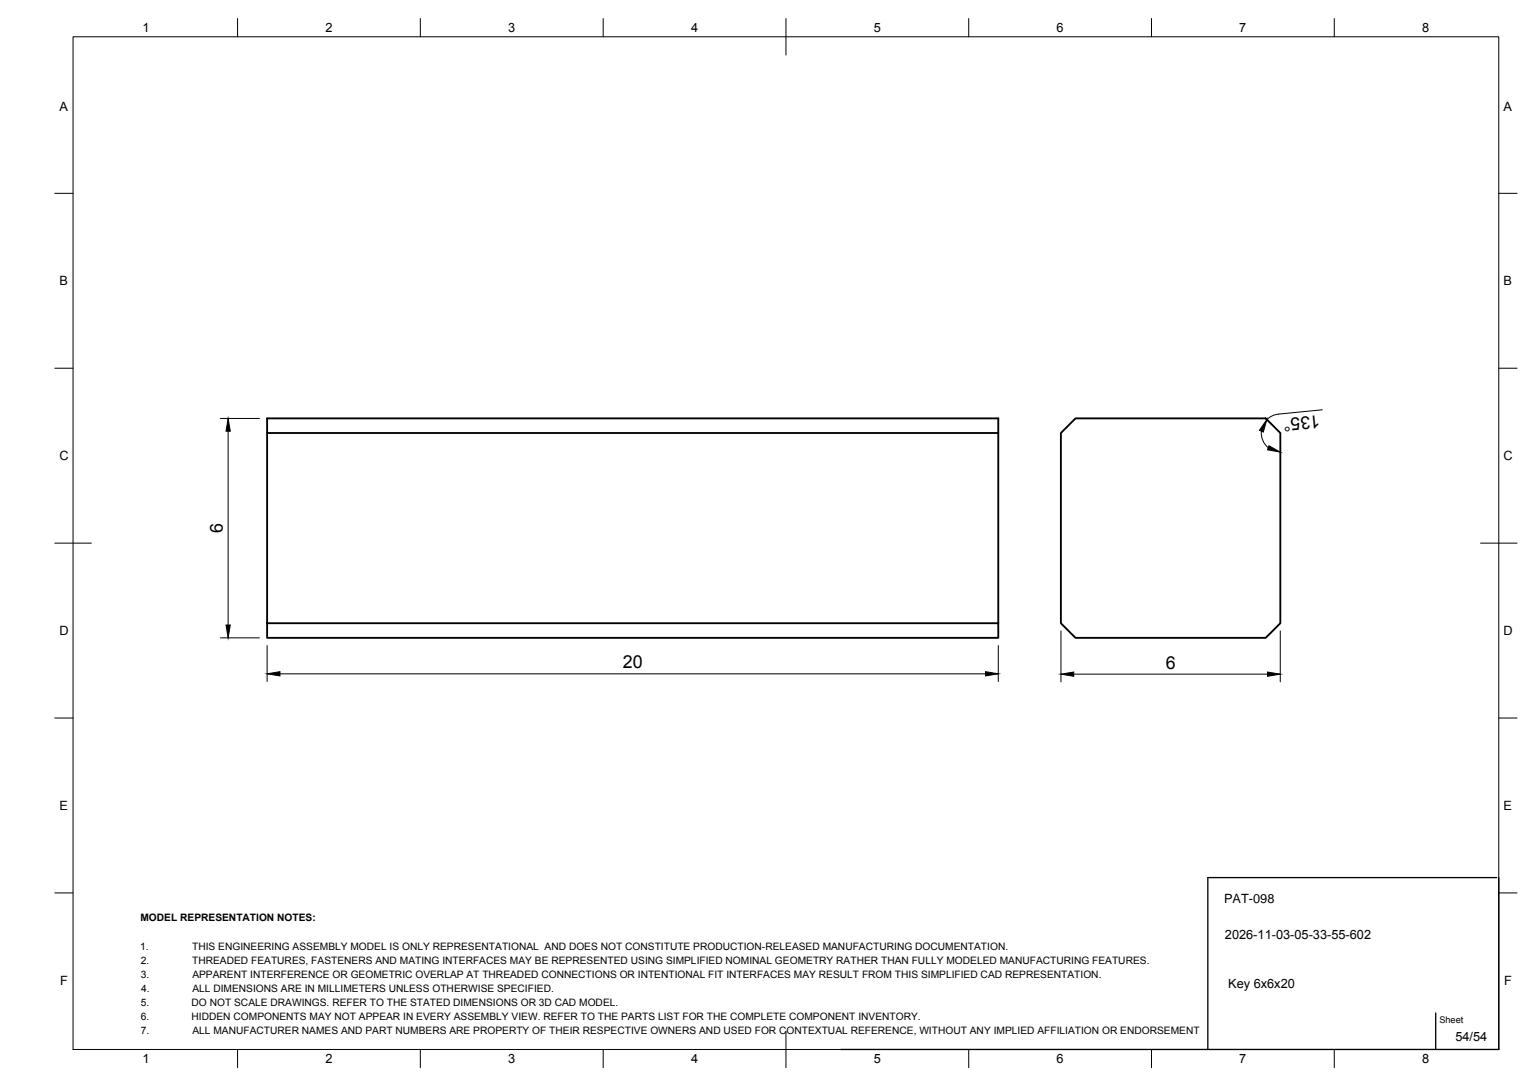
ISO-10303-21;
HEADER;
/* Generated by software containing ST-Developer
 * from STEP Tools, Inc. (www.steptools.com) 
 */

FILE_DESCRIPTION(
/* description */ ('Spring compression tester'),
/* implementation_level */ '2;1');

FILE_NAME(
/* name */ 'Key 6x6x20.step',
/* time_stamp */ '2026-10-28T03:24:11-07:00',
/* author */ (''),
/* organization */ (''),
/* preprocessor_version */ 'ST-DEVELOPER v20.2',
/* originating_system */ 'Autodesk Translation Framework v15.17.0.0',
/* authorisation */ '');

FILE_SCHEMA (('AUTOMOTIVE_DESIGN { 1 0 10303 214 3 1 1 }'));
ENDSEC;

DATA;
#10=MECHANICAL_DESIGN_GEOMETRIC_PRESENTATION_REPRESENTATION('',(#1175),#43521);
#1040=SHAPE_REPRESENTATION_RELATIONSHIP('SRR','None',#43857,#1100);
#1100=ADVANCED_BREP_SHAPE_REPRESENTATION('',(#1244),#43517);
#1175=STYLED_ITEM('',(#44202),#1244);
#1244=MANIFOLD_SOLID_BREP('Body1',#18618);
#2138=PLANE('',#21120);
#2139=PLANE('',#21121);
#2140=PLANE('',#21122);
#2141=PLANE('',#21123);
#2142=PLANE('',#21124);
#2143=PLANE('',#21125);
#2144=PLANE('',#21126);
#2145=PLANE('',#21127);
#2146=PLANE('',#21128);
#2147=PLANE('',#21129);
#3174=FACE_OUTER_BOUND('',#4559,.T.);
#3175=FACE_OUTER_BOUND('',#4560,.T.);
#3176=FACE_OUTER_BOUND('',#4561,.T.);
#3177=FACE_OUTER_BOUND('',#4562,.T.);
#3178=FACE_OUTER_BOUND('',#4563,.T.);
#3179=FACE_OUTER_BOUND('',#4564,.T.);
#3180=FACE_OUTER_BOUND('',#4565,.T.);
#3181=FACE_OUTER_BOUND('',#4566,.T.);
#3182=FACE_OUTER_BOUND('',#4567,.T.);
#3183=FACE_OUTER_BOUND('',#4568,.T.);
#4559=EDGE_LOOP('',(#16931,#16932,#16933,#16934,#16935,#16936,#16937,#16938));
#4560=EDGE_LOOP('',(#16939,#16940,#16941,#16942));
#4561=EDGE_LOOP('',(#16943,#16944,#16945,#16946));
#4562=EDGE_LOOP('',(#16947,#16948,#16949,#16950));
#4563=EDGE_LOOP('',(#16951,#16952,#16953,#16954));
#4564=EDGE_LOOP('',(#16955,#16956,#16957,#16958,#16959,#16960,#16961,#16962));
#4565=EDGE_LOOP('',(#16963,#16964,#16965,#16966));
#4566=EDGE_LOOP('',(#16967,#16968,#16969,#16970));
#4567=EDGE_LOOP('',(#16971,#16972,#16973,#16974));
#4568=EDGE_LOOP('',(#16975,#16976,#16977,#16978));
#5967=LINE('',#43186,#7399);
#5968=LINE('',#43188,#7400);
#5969=LINE('',#43190,#7401);
#5970=LINE('',#43192,#7402);
#5971=LINE('',#43194,#7403);
#5972=LINE('',#43196,#7404);
#5973=LINE('',#43198,#7405);
#5974=LINE('',#43199,#7406);
#5975=LINE('',#43202,#7407);
#5976=LINE('',#43204,#7408);
#5977=LINE('',#43205,#7409);
#5978=LINE('',#43208,#7410);
#5979=LINE('',#43209,#7411);
#5980=LINE('',#43212,#7412);
#5981=LINE('',#43213,#7413);
#5982=LINE('',#43216,#7414);
#5983=LINE('',#43217,#7415);
#5984=LINE('',#43221,#7416);
#5985=LINE('',#43222,#7417);
#5986=LINE('',#43224,#7418);
#5987=LINE('',#43225,#7419);
#5988=LINE('',#43227,#7420);
#5989=LINE('',#43229,#7421);
#5990=LINE('',#43231,#7422);
#7399=VECTOR('',#26231,1.);
#7400=VECTOR('',#26232,1.);
#7401=VECTOR('',#26233,1.);
#7402=VECTOR('',#26234,1.);
#7403=VECTOR('',#26235,1.);
#7404=VECTOR('',#26236,1.);
#7405=VECTOR('',#26237,1.);
#7406=VECTOR('',#26238,1.);
#7407=VECTOR('',#26241,1.);
#7408=VECTOR('',#26242,1.);
#7409=VECTOR('',#26243,1.);
#7410=VECTOR('',#26246,1.);
#7411=VECTOR('',#26247,1.);
#7412=VECTOR('',#26250,1.);
#7413=VECTOR('',#26251,1.);
#7414=VECTOR('',#26254,1.);
#7415=VECTOR('',#26255,1.);
#7416=VECTOR('',#26258,1.);
#7417=VECTOR('',#26259,1.);
#7418=VECTOR('',#26260,1.);
#7419=VECTOR('',#26261,1.);
#7420=VECTOR('',#26264,1.);
#7421=VECTOR('',#26267,1.);
#7422=VECTOR('',#26270,1.);
#9717=VERTEX_POINT('',#43184);
#9718=VERTEX_POINT('',#43185);
#9719=VERTEX_POINT('',#43187);
#9720=VERTEX_POINT('',#43189);
#9721=VERTEX_POINT('',#43191);
#9722=VERTEX_POINT('',#43193);
#9723=VERTEX_POINT('',#43195);
#9724=VERTEX_POINT('',#43197);
#9725=VERTEX_POINT('',#43201);
#9726=VERTEX_POINT('',#43203);
#9727=VERTEX_POINT('',#43207);
#9728=VERTEX_POINT('',#43211);
#9729=VERTEX_POINT('',#43215);
#9730=VERTEX_POINT('',#43219);
#9731=VERTEX_POINT('',#43220);
#9732=VERTEX_POINT('',#43223);
#12130=EDGE_CURVE('',#9717,#9718,#5967,.T.);
#12131=EDGE_CURVE('',#9719,#9717,#5968,.T.);
#12132=EDGE_CURVE('',#9720,#9719,#5969,.T.);
#12133=EDGE_CURVE('',#9721,#9720,#5970,.T.);
#12134=EDGE_CURVE('',#9722,#9721,#5971,.T.);
#12135=EDGE_CURVE('',#9723,#9722,#5972,.T.);
#12136=EDGE_CURVE('',#9724,#9723,#5973,.T.);
#12137=EDGE_CURVE('',#9718,#9724,#5974,.T.);
#12138=EDGE_CURVE('',#9721,#9725,#5975,.T.);
#12139=EDGE_CURVE('',#9725,#9726,#5976,.T.);
#12140=EDGE_CURVE('',#9726,#9722,#5977,.T.);
#12141=EDGE_CURVE('',#9727,#9720,#5978,.T.);
#12142=EDGE_CURVE('',#9727,#9725,#5979,.T.);
#12143=EDGE_CURVE('',#9719,#9728,#5980,.T.);
#12144=EDGE_CURVE('',#9728,#9727,#5981,.T.);
#12145=EDGE_CURVE('',#9729,#9717,#5982,.T.);
#12146=EDGE_CURVE('',#9729,#9728,#5983,.T.);
#12147=EDGE_CURVE('',#9730,#9731,#5984,.T.);
#12148=EDGE_CURVE('',#9726,#9730,#5985,.T.);
#12149=EDGE_CURVE('',#9732,#9729,#5986,.T.);
#12150=EDGE_CURVE('',#9731,#9732,#5987,.T.);
#12151=EDGE_CURVE('',#9723,#9730,#5988,.T.);
#12152=EDGE_CURVE('',#9718,#9732,#5989,.T.);
#12153=EDGE_CURVE('',#9731,#9724,#5990,.T.);
#16931=ORIENTED_EDGE('',*,*,#12130,.F.);
#16932=ORIENTED_EDGE('',*,*,#12131,.F.);
#16933=ORIENTED_EDGE('',*,*,#12132,.F.);
#16934=ORIENTED_EDGE('',*,*,#12133,.F.);
#16935=ORIENTED_EDGE('',*,*,#12134,.F.);
#16936=ORIENTED_EDGE('',*,*,#12135,.F.);
#16937=ORIENTED_EDGE('',*,*,#12136,.F.);
#16938=ORIENTED_EDGE('',*,*,#12137,.F.);
#16939=ORIENTED_EDGE('',*,*,#12134,.T.);
#16940=ORIENTED_EDGE('',*,*,#12138,.T.);
#16941=ORIENTED_EDGE('',*,*,#12139,.T.);
#16942=ORIENTED_EDGE('',*,*,#12140,.T.);
#16943=ORIENTED_EDGE('',*,*,#12133,.T.);
#16944=ORIENTED_EDGE('',*,*,#12141,.F.);
#16945=ORIENTED_EDGE('',*,*,#12142,.T.);
#16946=ORIENTED_EDGE('',*,*,#12138,.F.);
#16947=ORIENTED_EDGE('',*,*,#12132,.T.);
#16948=ORIENTED_EDGE('',*,*,#12143,.T.);
#16949=ORIENTED_EDGE('',*,*,#12144,.T.);
#16950=ORIENTED_EDGE('',*,*,#12141,.T.);
#16951=ORIENTED_EDGE('',*,*,#12131,.T.);
#16952=ORIENTED_EDGE('',*,*,#12145,.F.);
#16953=ORIENTED_EDGE('',*,*,#12146,.T.);
#16954=ORIENTED_EDGE('',*,*,#12143,.F.);
#16955=ORIENTED_EDGE('',*,*,#12147,.F.);
#16956=ORIENTED_EDGE('',*,*,#12148,.F.);
#16957=ORIENTED_EDGE('',*,*,#12139,.F.);
#16958=ORIENTED_EDGE('',*,*,#12142,.F.);
#16959=ORIENTED_EDGE('',*,*,#12144,.F.);
#16960=ORIENTED_EDGE('',*,*,#12146,.F.);
#16961=ORIENTED_EDGE('',*,*,#12149,.F.);
#16962=ORIENTED_EDGE('',*,*,#12150,.F.);
#16963=ORIENTED_EDGE('',*,*,#12135,.T.);
#16964=ORIENTED_EDGE('',*,*,#12140,.F.);
#16965=ORIENTED_EDGE('',*,*,#12148,.T.);
#16966=ORIENTED_EDGE('',*,*,#12151,.F.);
#16967=ORIENTED_EDGE('',*,*,#12130,.T.);
#16968=ORIENTED_EDGE('',*,*,#12152,.T.);
#16969=ORIENTED_EDGE('',*,*,#12149,.T.);
#16970=ORIENTED_EDGE('',*,*,#12145,.T.);
#16971=ORIENTED_EDGE('',*,*,#12136,.T.);
#16972=ORIENTED_EDGE('',*,*,#12151,.T.);
#16973=ORIENTED_EDGE('',*,*,#12147,.T.);
#16974=ORIENTED_EDGE('',*,*,#12153,.T.);
#16975=ORIENTED_EDGE('',*,*,#12137,.T.);
#16976=ORIENTED_EDGE('',*,*,#12153,.F.);
#16977=ORIENTED_EDGE('',*,*,#12150,.T.);
#16978=ORIENTED_EDGE('',*,*,#12152,.F.);
#18498=ADVANCED_FACE('',(#3174),#2138,.F.);
#18499=ADVANCED_FACE('',(#3175),#2139,.T.);
#18500=ADVANCED_FACE('',(#3176),#2140,.T.);
#18501=ADVANCED_FACE('',(#3177),#2141,.T.);
#18502=ADVANCED_FACE('',(#3178),#2142,.T.);
#18503=ADVANCED_FACE('',(#3179),#2143,.T.);
#18504=ADVANCED_FACE('',(#3180),#2144,.F.);
#18505=ADVANCED_FACE('',(#3181),#2145,.T.);
#18506=ADVANCED_FACE('',(#3182),#2146,.T.);
#18507=ADVANCED_FACE('',(#3183),#2147,.T.);
#18618=CLOSED_SHELL('',(#18498,#18499,#18500,#18501,#18502,#18503,#18504,
#18505,#18506,#18507));
#21119=AXIS2_PLACEMENT_3D('',#43182,#26227,#26228);
#21120=AXIS2_PLACEMENT_3D('',#43183,#26229,#26230);
#21121=AXIS2_PLACEMENT_3D('',#43200,#26239,#26240);
#21122=AXIS2_PLACEMENT_3D('',#43206,#26244,#26245);
#21123=AXIS2_PLACEMENT_3D('',#43210,#26248,#26249);
#21124=AXIS2_PLACEMENT_3D('',#43214,#26252,#26253);
#21125=AXIS2_PLACEMENT_3D('',#43218,#26256,#26257);
#21126=AXIS2_PLACEMENT_3D('',#43226,#26262,#26263);
#21127=AXIS2_PLACEMENT_3D('',#43228,#26265,#26266);
#21128=AXIS2_PLACEMENT_3D('',#43230,#26268,#26269);
#21129=AXIS2_PLACEMENT_3D('',#43232,#26271,#26272);
#26227=DIRECTION('axis',(0.,0.,1.));
#26228=DIRECTION('refdir',(1.,0.,0.));
#26229=DIRECTION('center_axis',(1.,0.,0.));
#26230=DIRECTION('ref_axis',(0.,0.,-1.));
#26231=DIRECTION('',(0.,-0.707106781186547,-0.707106781186548));
#26232=DIRECTION('',(0.,-1.,0.));
#26233=DIRECTION('',(0.,-0.707106781186547,0.707106781186548));
#26234=DIRECTION('',(0.,0.,1.));
#26235=DIRECTION('',(0.,0.707106781186547,0.707106781186548));
#26236=DIRECTION('',(0.,1.,0.));
#26237=DIRECTION('',(0.,0.707106781186547,-0.707106781186548));
#26238=DIRECTION('',(0.,0.,-1.));
#26239=DIRECTION('center_axis',(0.,0.707106781186548,-0.707106781186547));
#26240=DIRECTION('ref_axis',(-1.,0.,0.));
#26241=DIRECTION('',(1.,0.,0.));
#26242=DIRECTION('',(0.,-0.707106781186547,-0.707106781186548));
#26243=DIRECTION('',(-1.,0.,0.));
#26244=DIRECTION('center_axis',(0.,1.,0.));
#26245=DIRECTION('ref_axis',(-1.,0.,0.));
#26246=DIRECTION('',(-1.,0.,0.));
#26247=DIRECTION('',(0.,0.,-1.));
#26248=DIRECTION('center_axis',(0.,0.707106781186548,0.707106781186547));
#26249=DIRECTION('ref_axis',(1.,0.,0.));
#26250=DIRECTION('',(1.,0.,0.));
#26251=DIRECTION('',(0.,0.707106781186547,-0.707106781186548));
#26252=DIRECTION('center_axis',(0.,0.,1.));
#26253=DIRECTION('ref_axis',(1.,0.,0.));
#26254=DIRECTION('',(-1.,0.,0.));
#26255=DIRECTION('',(0.,1.,0.));
#26256=DIRECTION('center_axis',(1.,0.,0.));
#26257=DIRECTION('ref_axis',(0.,0.,-1.));
#26258=DIRECTION('',(0.,-0.707106781186547,0.707106781186548));
#26259=DIRECTION('',(0.,-1.,0.));
#26260=DIRECTION('',(0.,0.707106781186547,0.707106781186548));
#26261=DIRECTION('',(0.,0.,1.));
#26262=DIRECTION('center_axis',(0.,0.,1.));
#26263=DIRECTION('ref_axis',(1.,0.,0.));
#26264=DIRECTION('',(1.,0.,0.));
#26265=DIRECTION('center_axis',(0.,-0.707106781186548,0.707106781186547));
#26266=DIRECTION('ref_axis',(1.,0.,0.));
#26267=DIRECTION('',(1.,0.,0.));
#26268=DIRECTION('center_axis',(0.,-0.707106781186548,-0.707106781186547));
#26269=DIRECTION('ref_axis',(-1.,0.,0.));
#26270=DIRECTION('',(-1.,0.,0.));
#26271=DIRECTION('center_axis',(0.,-1.,0.));
#26272=DIRECTION('ref_axis',(1.,0.,0.));
#43182=CARTESIAN_POINT('',(0.,0.,0.));
#43183=CARTESIAN_POINT('Origin',(-1.,0.,0.35));
#43184=CARTESIAN_POINT('',(-1.,-0.26,0.6));
#43185=CARTESIAN_POINT('',(-1.,-0.3,0.56));
#43186=CARTESIAN_POINT('',(-1.,-0.2675,0.5925));
#43187=CARTESIAN_POINT('',(-1.,0.26,0.6));
#43188=CARTESIAN_POINT('',(-1.,0.,0.6));
#43189=CARTESIAN_POINT('',(-1.,0.3,0.56));
#43190=CARTESIAN_POINT('',(-1.,0.2675,0.5925));
#43191=CARTESIAN_POINT('',(-1.,0.3,0.04));
#43192=CARTESIAN_POINT('',(-1.,0.3,0.175));
#43193=CARTESIAN_POINT('',(-1.,0.26,0.));
#43194=CARTESIAN_POINT('',(-1.,0.2925,0.0325));
#43195=CARTESIAN_POINT('',(-1.,-0.26,0.));
#43196=CARTESIAN_POINT('',(-1.,0.,0.));
#43197=CARTESIAN_POINT('',(-1.,-0.3,0.04));
#43198=CARTESIAN_POINT('',(-1.,-0.2925,0.0325));
#43199=CARTESIAN_POINT('',(-1.,-0.3,0.175));
#43200=CARTESIAN_POINT('Origin',(0.75,0.28,0.02));
#43201=CARTESIAN_POINT('',(1.,0.3,0.04));
#43202=CARTESIAN_POINT('',(0.75,0.3,0.04));
#43203=CARTESIAN_POINT('',(1.,0.26,0.));
#43204=CARTESIAN_POINT('',(1.,0.2925,0.0325));
#43205=CARTESIAN_POINT('',(0.75,0.26,0.));
#43206=CARTESIAN_POINT('Origin',(1.5,0.3,0.));
#43207=CARTESIAN_POINT('',(1.,0.3,0.56));
#43208=CARTESIAN_POINT('',(0.75,0.3,0.56));
#43209=CARTESIAN_POINT('',(1.,0.3,0.175));
#43210=CARTESIAN_POINT('Origin',(0.75,0.28,0.58));
#43211=CARTESIAN_POINT('',(1.,0.26,0.6));
#43212=CARTESIAN_POINT('',(0.75,0.26,0.6));
#43213=CARTESIAN_POINT('',(1.,0.2675,0.5925));
#43214=CARTESIAN_POINT('Origin',(0.,0.,0.6));
#43215=CARTESIAN_POINT('',(1.,-0.26,0.6));
#43216=CARTESIAN_POINT('',(-0.75,-0.26,0.6));
#43217=CARTESIAN_POINT('',(1.,0.,0.6));
#43218=CARTESIAN_POINT('Origin',(1.,0.,0.35));
#43219=CARTESIAN_POINT('',(1.,-0.26,0.));
#43220=CARTESIAN_POINT('',(1.,-0.3,0.04));
#43221=CARTESIAN_POINT('',(1.,-0.2925,0.0325));
#43222=CARTESIAN_POINT('',(1.,0.,0.));
#43223=CARTESIAN_POINT('',(1.,-0.3,0.56));
#43224=CARTESIAN_POINT('',(1.,-0.2675,0.5925));
#43225=CARTESIAN_POINT('',(1.,-0.3,0.175));
#43226=CARTESIAN_POINT('Origin',(0.,0.,0.));
#43227=CARTESIAN_POINT('',(-0.75,-0.26,0.));
#43228=CARTESIAN_POINT('Origin',(-0.75,-0.28,0.58));
#43229=CARTESIAN_POINT('',(-0.75,-0.3,0.56));
#43230=CARTESIAN_POINT('Origin',(-0.75,-0.28,0.02));
#43231=CARTESIAN_POINT('',(-0.75,-0.3,0.04));
#43232=CARTESIAN_POINT('Origin',(-1.5,-0.3,0.));
#43449=UNCERTAINTY_MEASURE_WITH_UNIT(LENGTH_MEASURE(0.001),#43522,
'DISTANCE_ACCURACY_VALUE',
'Maximum model space distance between geometric entities at asserted c
onnectivities');
#43453=UNCERTAINTY_MEASURE_WITH_UNIT(LENGTH_MEASURE(0.001),#43522,
'DISTANCE_ACCURACY_VALUE',
'Maximum model space distance between geometric entities at asserted c
onnectivities');
#43517=(
GEOMETRIC_REPRESENTATION_CONTEXT(3)
GLOBAL_UNCERTAINTY_ASSIGNED_CONTEXT((#43449))
GLOBAL_UNIT_ASSIGNED_CONTEXT((#43522,#43524,#43525))
REPRESENTATION_CONTEXT('','3D')
);
#43521=(
GEOMETRIC_REPRESENTATION_CONTEXT(3)
GLOBAL_UNCERTAINTY_ASSIGNED_CONTEXT((#43453))
GLOBAL_UNIT_ASSIGNED_CONTEXT((#43522,#43524,#43525))
REPRESENTATION_CONTEXT('','3D')
);
#43522=(
LENGTH_UNIT()
NAMED_UNIT(*)
SI_UNIT(.CENTI.,.METRE.)
);
#43524=(
NAMED_UNIT(*)
PLANE_ANGLE_UNIT()
SI_UNIT($,.RADIAN.)
);
#43525=(
NAMED_UNIT(*)
SI_UNIT($,.STERADIAN.)
SOLID_ANGLE_UNIT()
);
#43589=SHAPE_DEFINITION_REPRESENTATION(#43776,#43857);
#43776=PRODUCT_DEFINITION_SHAPE('',$,#43925);
#43857=SHAPE_REPRESENTATION('',(#21119),#43517);
#43861=PRODUCT_DEFINITION_CONTEXT('part definition',#44064,'design');
#43925=PRODUCT_DEFINITION('Key 6x6x20','Key 6x6x20',#43992,#43861);
#43992=PRODUCT_DEFINITION_FORMATION('',$,#44129);
#44064=APPLICATION_CONTEXT(
'Core Data for Automotive Mechanical Design Process');
#44065=PRODUCT_CONTEXT('part definition',#44064,'mechanical');
#44129=PRODUCT('Key 6x6x20','Key 6x6x20','Key 6x6x20',(#44065));
#44196=COLOUR_RGB('Grey',0.48,0.52,0.57);
#44197=FILL_AREA_STYLE_COLOUR('',#44196);
#44198=FILL_AREA_STYLE('',(#44197));
#44199=SURFACE_STYLE_FILL_AREA(#44198);
#44200=SURFACE_SIDE_STYLE('',(#44199));
#44201=SURFACE_STYLE_USAGE(.BOTH.,#44200);
#44202=PRESENTATION_STYLE_ASSIGNMENT((#44201));
ENDSEC;
END-ISO-10303-21;
